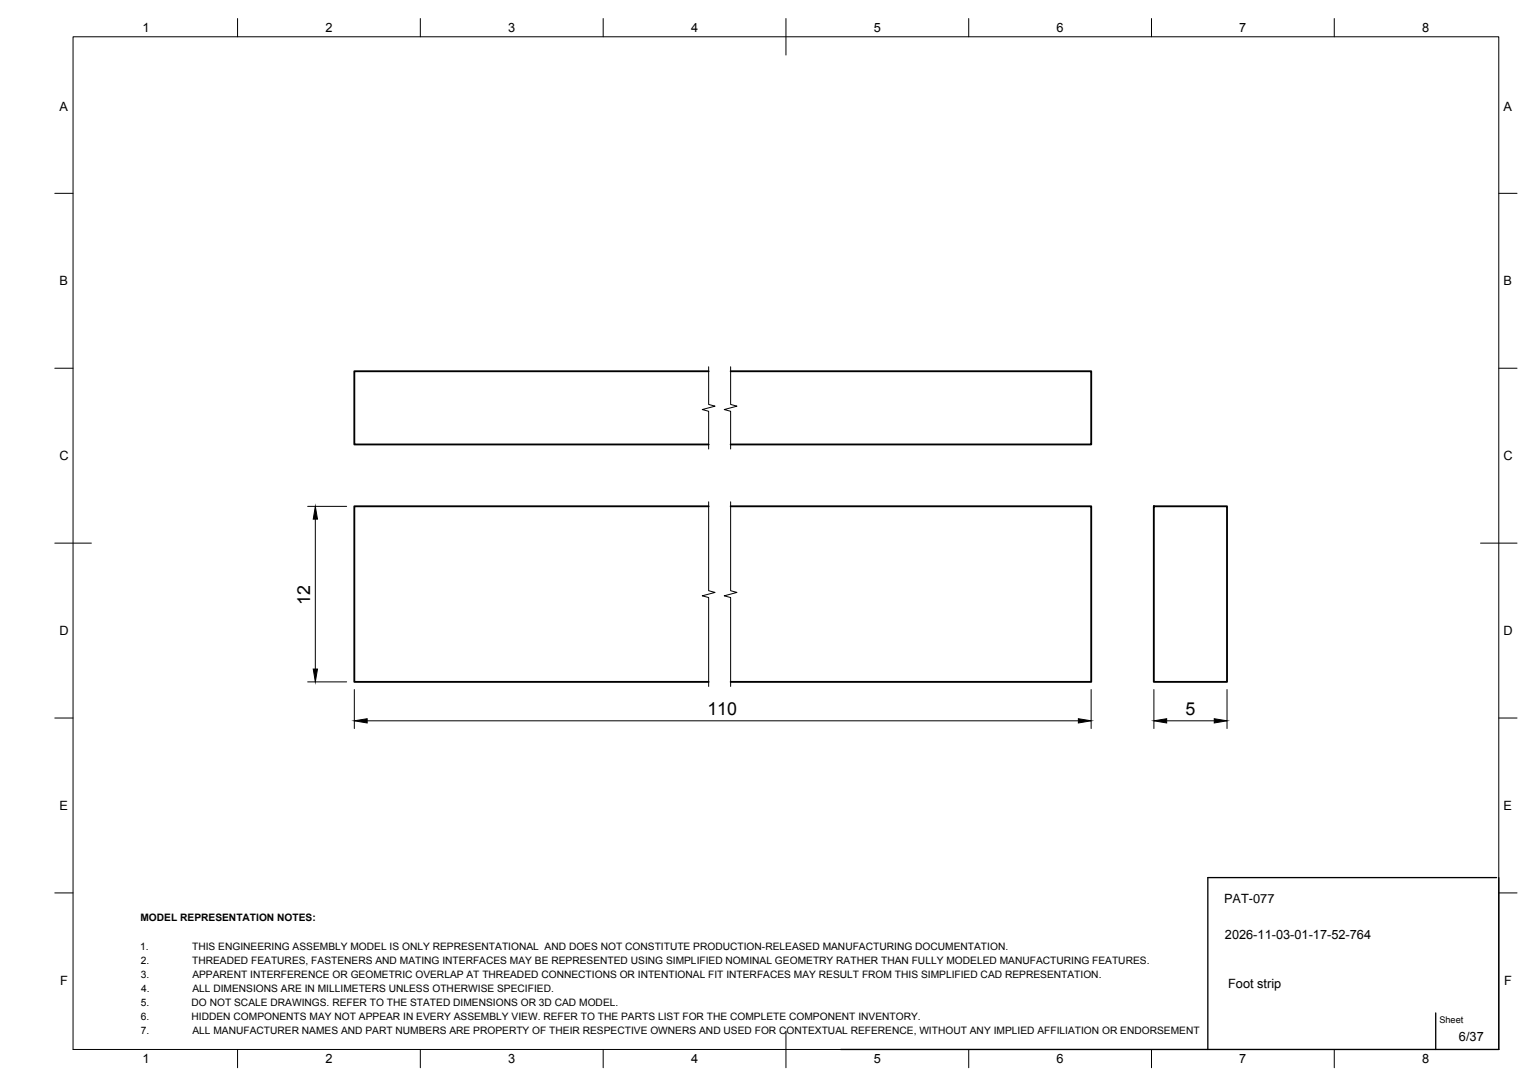
ISO-10303-21;
HEADER;
/* Generated by software containing ST-Developer
 * from STEP Tools, Inc. (www.steptools.com) 
 */

FILE_DESCRIPTION(
/* description */ ('Pallet stop with pneumatic fitting'),
/* implementation_level */ '2;1');

FILE_NAME(
/* name */ 'Foot strip.step',
/* time_stamp */ '2026-10-27T10:51:41-07:00',
/* author */ (''),
/* organization */ (''),
/* preprocessor_version */ 'ST-DEVELOPER v20.2',
/* originating_system */ 'Autodesk Translation Framework v15.17.0.0',
/* authorisation */ '');

FILE_SCHEMA (('AUTOMOTIVE_DESIGN { 1 0 10303 214 3 1 1 }'));
ENDSEC;

DATA;
#10=MECHANICAL_DESIGN_GEOMETRIC_PRESENTATION_REPRESENTATION('',(#358),#10265);
#294=SHAPE_REPRESENTATION_RELATIONSHIP('SRR','None',#10407,#326);
#326=ADVANCED_BREP_SHAPE_REPRESENTATION('',(#390),#10231);
#358=STYLED_ITEM('',(#10641),#390);
#390=MANIFOLD_SOLID_BREP('Body1',#5046);
#551=PLANE('',#5469);
#552=PLANE('',#5470);
#553=PLANE('',#5471);
#554=PLANE('',#5472);
#555=PLANE('',#5473);
#556=PLANE('',#5474);
#751=FACE_OUTER_BOUND('',#1083,.T.);
#752=FACE_OUTER_BOUND('',#1084,.T.);
#753=FACE_OUTER_BOUND('',#1085,.T.);
#754=FACE_OUTER_BOUND('',#1086,.T.);
#755=FACE_OUTER_BOUND('',#1087,.T.);
#756=FACE_OUTER_BOUND('',#1088,.T.);
#1083=EDGE_LOOP('',(#3488,#3489,#3490,#3491));
#1084=EDGE_LOOP('',(#3492,#3493,#3494,#3495));
#1085=EDGE_LOOP('',(#3496,#3497,#3498,#3499));
#1086=EDGE_LOOP('',(#3500,#3501,#3502,#3503));
#1087=EDGE_LOOP('',(#3504,#3505,#3506,#3507));
#1088=EDGE_LOOP('',(#3508,#3509,#3510,#3511));
#1511=LINE('',#7825,#1846);
#1512=LINE('',#7827,#1847);
#1513=LINE('',#7829,#1848);
#1514=LINE('',#7830,#1849);
#1515=LINE('',#7833,#1850);
#1516=LINE('',#7835,#1851);
#1517=LINE('',#7836,#1852);
#1518=LINE('',#7839,#1853);
#1519=LINE('',#7841,#1854);
#1520=LINE('',#7842,#1855);
#1521=LINE('',#7844,#1856);
#1522=LINE('',#7845,#1857);
#1846=VECTOR('',#6186,1.);
#1847=VECTOR('',#6187,1.);
#1848=VECTOR('',#6188,1.);
#1849=VECTOR('',#6189,1.);
#1850=VECTOR('',#6192,1.);
#1851=VECTOR('',#6193,1.);
#1852=VECTOR('',#6194,1.);
#1853=VECTOR('',#6197,1.);
#1854=VECTOR('',#6198,1.);
#1855=VECTOR('',#6199,1.);
#1856=VECTOR('',#6202,1.);
#1857=VECTOR('',#6203,1.);
#2433=VERTEX_POINT('',#7823);
#2434=VERTEX_POINT('',#7824);
#2435=VERTEX_POINT('',#7826);
#2436=VERTEX_POINT('',#7828);
#2437=VERTEX_POINT('',#7832);
#2438=VERTEX_POINT('',#7834);
#2439=VERTEX_POINT('',#7838);
#2440=VERTEX_POINT('',#7840);
#2843=EDGE_CURVE('',#2433,#2434,#1511,.T.);
#2844=EDGE_CURVE('',#2434,#2435,#1512,.T.);
#2845=EDGE_CURVE('',#2436,#2435,#1513,.T.);
#2846=EDGE_CURVE('',#2433,#2436,#1514,.T.);
#2847=EDGE_CURVE('',#2437,#2433,#1515,.T.);
#2848=EDGE_CURVE('',#2438,#2436,#1516,.T.);
#2849=EDGE_CURVE('',#2437,#2438,#1517,.T.);
#2850=EDGE_CURVE('',#2439,#2437,#1518,.T.);
#2851=EDGE_CURVE('',#2440,#2438,#1519,.T.);
#2852=EDGE_CURVE('',#2439,#2440,#1520,.T.);
#2853=EDGE_CURVE('',#2434,#2439,#1521,.T.);
#2854=EDGE_CURVE('',#2435,#2440,#1522,.T.);
#3488=ORIENTED_EDGE('',*,*,#2843,.T.);
#3489=ORIENTED_EDGE('',*,*,#2844,.T.);
#3490=ORIENTED_EDGE('',*,*,#2845,.F.);
#3491=ORIENTED_EDGE('',*,*,#2846,.F.);
#3492=ORIENTED_EDGE('',*,*,#2847,.T.);
#3493=ORIENTED_EDGE('',*,*,#2846,.T.);
#3494=ORIENTED_EDGE('',*,*,#2848,.F.);
#3495=ORIENTED_EDGE('',*,*,#2849,.F.);
#3496=ORIENTED_EDGE('',*,*,#2850,.T.);
#3497=ORIENTED_EDGE('',*,*,#2849,.T.);
#3498=ORIENTED_EDGE('',*,*,#2851,.F.);
#3499=ORIENTED_EDGE('',*,*,#2852,.F.);
#3500=ORIENTED_EDGE('',*,*,#2853,.T.);
#3501=ORIENTED_EDGE('',*,*,#2852,.T.);
#3502=ORIENTED_EDGE('',*,*,#2854,.F.);
#3503=ORIENTED_EDGE('',*,*,#2844,.F.);
#3504=ORIENTED_EDGE('',*,*,#2854,.T.);
#3505=ORIENTED_EDGE('',*,*,#2851,.T.);
#3506=ORIENTED_EDGE('',*,*,#2848,.T.);
#3507=ORIENTED_EDGE('',*,*,#2845,.T.);
#3508=ORIENTED_EDGE('',*,*,#2853,.F.);
#3509=ORIENTED_EDGE('',*,*,#2843,.F.);
#3510=ORIENTED_EDGE('',*,*,#2847,.F.);
#3511=ORIENTED_EDGE('',*,*,#2850,.F.);
#4746=ADVANCED_FACE('',(#751),#551,.T.);
#4747=ADVANCED_FACE('',(#752),#552,.T.);
#4748=ADVANCED_FACE('',(#753),#553,.T.);
#4749=ADVANCED_FACE('',(#754),#554,.T.);
#4750=ADVANCED_FACE('',(#755),#555,.T.);
#4751=ADVANCED_FACE('',(#756),#556,.F.);
#5046=CLOSED_SHELL('',(#4746,#4747,#4748,#4749,#4750,#4751));
#5468=AXIS2_PLACEMENT_3D('',#7821,#6182,#6183);
#5469=AXIS2_PLACEMENT_3D('',#7822,#6184,#6185);
#5470=AXIS2_PLACEMENT_3D('',#7831,#6190,#6191);
#5471=AXIS2_PLACEMENT_3D('',#7837,#6195,#6196);
#5472=AXIS2_PLACEMENT_3D('',#7843,#6200,#6201);
#5473=AXIS2_PLACEMENT_3D('',#7846,#6204,#6205);
#5474=AXIS2_PLACEMENT_3D('',#7847,#6206,#6207);
#6182=DIRECTION('axis',(0.,0.,1.));
#6183=DIRECTION('refdir',(1.,0.,0.));
#6184=DIRECTION('center_axis',(0.,1.,0.));
#6185=DIRECTION('ref_axis',(-1.,0.,0.));
#6186=DIRECTION('',(-1.,0.,0.));
#6187=DIRECTION('',(0.,0.,1.));
#6188=DIRECTION('',(-1.,0.,0.));
#6189=DIRECTION('',(0.,0.,1.));
#6190=DIRECTION('center_axis',(1.,0.,0.));
#6191=DIRECTION('ref_axis',(0.,1.,0.));
#6192=DIRECTION('',(0.,1.,0.));
#6193=DIRECTION('',(0.,1.,0.));
#6194=DIRECTION('',(0.,0.,1.));
#6195=DIRECTION('center_axis',(0.,-1.,0.));
#6196=DIRECTION('ref_axis',(1.,0.,0.));
#6197=DIRECTION('',(1.,0.,0.));
#6198=DIRECTION('',(1.,0.,0.));
#6199=DIRECTION('',(0.,0.,1.));
#6200=DIRECTION('center_axis',(-1.,0.,0.));
#6201=DIRECTION('ref_axis',(0.,-1.,0.));
#6202=DIRECTION('',(0.,-1.,0.));
#6203=DIRECTION('',(0.,-1.,0.));
#6204=DIRECTION('center_axis',(0.,0.,1.));
#6205=DIRECTION('ref_axis',(1.,0.,0.));
#6206=DIRECTION('center_axis',(0.,0.,1.));
#6207=DIRECTION('ref_axis',(1.,0.,0.));
#7821=CARTESIAN_POINT('',(0.,0.,0.));
#7822=CARTESIAN_POINT('Origin',(-4.5,7.5,-2.2));
#7823=CARTESIAN_POINT('',(-4.5,7.5,-2.2));
#7824=CARTESIAN_POINT('',(-5.,7.5,-2.2));
#7825=CARTESIAN_POINT('',(-4.5,7.5,-2.2));
#7826=CARTESIAN_POINT('',(-5.,7.5,-1.));
#7827=CARTESIAN_POINT('',(-5.,7.5,-2.2));
#7828=CARTESIAN_POINT('',(-4.5,7.5,-1.));
#7829=CARTESIAN_POINT('',(-4.5,7.5,-1.));
#7830=CARTESIAN_POINT('',(-4.5,7.5,-2.2));
#7831=CARTESIAN_POINT('Origin',(-4.5,-3.5,-2.2));
#7832=CARTESIAN_POINT('',(-4.5,-3.5,-2.2));
#7833=CARTESIAN_POINT('',(-4.5,-3.5,-2.2));
#7834=CARTESIAN_POINT('',(-4.5,-3.5,-1.));
#7835=CARTESIAN_POINT('',(-4.5,-3.5,-1.));
#7836=CARTESIAN_POINT('',(-4.5,-3.5,-2.2));
#7837=CARTESIAN_POINT('Origin',(-5.,-3.5,-2.2));
#7838=CARTESIAN_POINT('',(-5.,-3.5,-2.2));
#7839=CARTESIAN_POINT('',(-5.,-3.5,-2.2));
#7840=CARTESIAN_POINT('',(-5.,-3.5,-1.));
#7841=CARTESIAN_POINT('',(-5.,-3.5,-1.));
#7842=CARTESIAN_POINT('',(-5.,-3.5,-2.2));
#7843=CARTESIAN_POINT('Origin',(-5.,7.5,-2.2));
#7844=CARTESIAN_POINT('',(-5.,7.5,-2.2));
#7845=CARTESIAN_POINT('',(-5.,7.5,-1.));
#7846=CARTESIAN_POINT('Origin',(-4.75,2.,-1.));
#7847=CARTESIAN_POINT('Origin',(-4.75,2.,-2.2));
#10193=UNCERTAINTY_MEASURE_WITH_UNIT(LENGTH_MEASURE(0.001),#10266,
'DISTANCE_ACCURACY_VALUE',
'Maximum model space distance between geometric entities at asserted c
onnectivities');
#10227=UNCERTAINTY_MEASURE_WITH_UNIT(LENGTH_MEASURE(0.001),#10266,
'DISTANCE_ACCURACY_VALUE',
'Maximum model space distance between geometric entities at asserted c
onnectivities');
#10231=(
GEOMETRIC_REPRESENTATION_CONTEXT(3)
GLOBAL_UNCERTAINTY_ASSIGNED_CONTEXT((#10193))
GLOBAL_UNIT_ASSIGNED_CONTEXT((#10266,#10268,#10269))
REPRESENTATION_CONTEXT('','3D')
);
#10265=(
GEOMETRIC_REPRESENTATION_CONTEXT(3)
GLOBAL_UNCERTAINTY_ASSIGNED_CONTEXT((#10227))
GLOBAL_UNIT_ASSIGNED_CONTEXT((#10266,#10268,#10269))
REPRESENTATION_CONTEXT('','3D')
);
#10266=(
LENGTH_UNIT()
NAMED_UNIT(*)
SI_UNIT(.CENTI.,.METRE.)
);
#10268=(
NAMED_UNIT(*)
PLANE_ANGLE_UNIT()
SI_UNIT($,.RADIAN.)
);
#10269=(
NAMED_UNIT(*)
SI_UNIT($,.STERADIAN.)
SOLID_ANGLE_UNIT()
);
#10273=SHAPE_DEFINITION_REPRESENTATION(#10310,#10407);
#10310=PRODUCT_DEFINITION_SHAPE('',$,#10445);
#10407=SHAPE_REPRESENTATION('',(#5468),#10231);
#10441=PRODUCT_DEFINITION_CONTEXT('part definition',#10554,'design');
#10445=PRODUCT_DEFINITION('Foot strip','Foot strip',#10482,#10441);
#10482=PRODUCT_DEFINITION_FORMATION('',$,#10559);
#10554=APPLICATION_CONTEXT(
'Core Data for Automotive Mechanical Design Process');
#10555=PRODUCT_CONTEXT('part definition',#10554,'mechanical');
#10559=PRODUCT('Foot strip','Foot strip','Foot strip',(#10555));
#10635=COLOUR_RGB('Light Blue',0.38,0.62,0.78);
#10636=FILL_AREA_STYLE_COLOUR('',#10635);
#10637=FILL_AREA_STYLE('',(#10636));
#10638=SURFACE_STYLE_FILL_AREA(#10637);
#10639=SURFACE_SIDE_STYLE('',(#10638));
#10640=SURFACE_STYLE_USAGE(.BOTH.,#10639);
#10641=PRESENTATION_STYLE_ASSIGNMENT((#10640));
ENDSEC;
END-ISO-10303-21;
